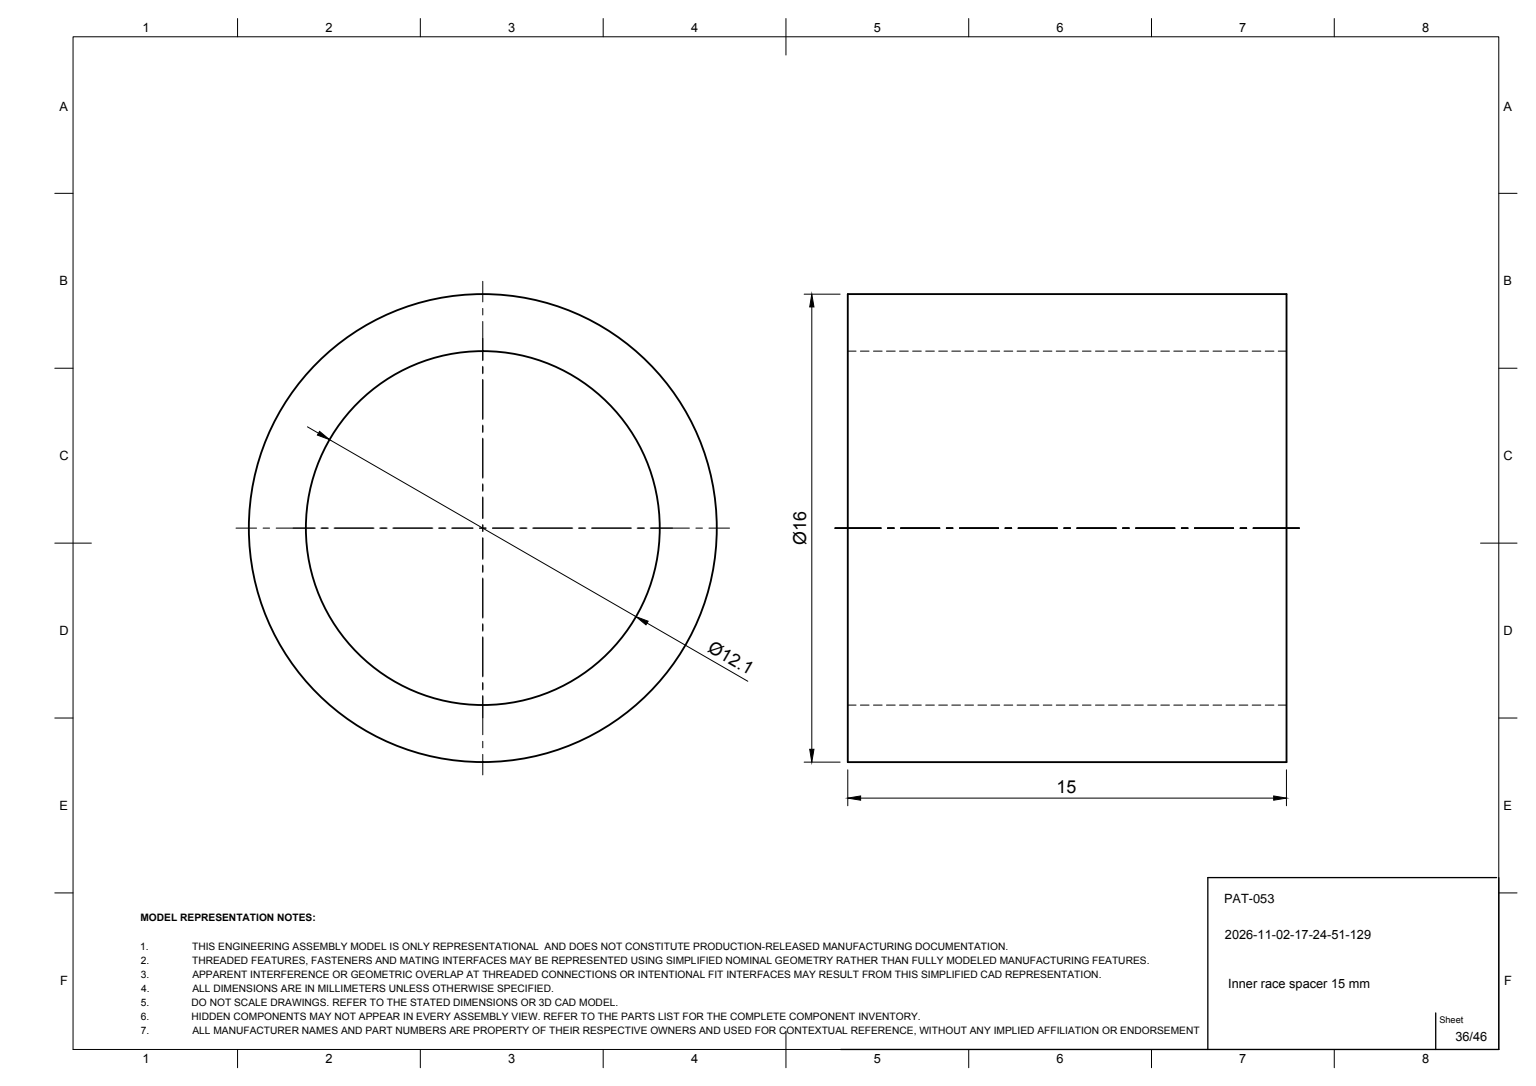
ISO-10303-21;
HEADER;
/* Generated by software containing ST-Developer
 * from STEP Tools, Inc. (www.steptools.com) 
 */

FILE_DESCRIPTION(
/* description */ ('Hand-operated arbor press'),
/* implementation_level */ '2;1');

FILE_NAME(
/* name */ 'Inner race spacer 15 mm.step',
/* time_stamp */ '2026-10-28T03:25:25-07:00',
/* author */ (''),
/* organization */ (''),
/* preprocessor_version */ 'ST-DEVELOPER v20.2',
/* originating_system */ 'Autodesk Translation Framework v15.17.0.0',
/* authorisation */ '');

FILE_SCHEMA (('AUTOMOTIVE_DESIGN { 1 0 10303 214 3 1 1 }'));
ENDSEC;

DATA;
#10=MECHANICAL_DESIGN_GEOMETRIC_PRESENTATION_REPRESENTATION('',(#621),#32751);
#530=SHAPE_REPRESENTATION_RELATIONSHIP('SRR','None',#32962,#572);
#572=ADVANCED_BREP_SHAPE_REPRESENTATION('',(#668),#32736);
#621=STYLED_ITEM('',(#33242),#668);
#668=MANIFOLD_SOLID_BREP('Body1',#12520);
#823=FACE_BOUND('',#2622,.T.);
#824=FACE_BOUND('',#2624,.T.);
#1208=PLANE('',#13838);
#1209=PLANE('',#13839);
#1795=FACE_OUTER_BOUND('',#2619,.T.);
#1796=FACE_OUTER_BOUND('',#2620,.T.);
#1797=FACE_OUTER_BOUND('',#2621,.T.);
#1798=FACE_OUTER_BOUND('',#2623,.T.);
#2619=EDGE_LOOP('',(#10800,#10801,#10802,#10803));
#2620=EDGE_LOOP('',(#10804,#10805,#10806,#10807));
#2621=EDGE_LOOP('',(#10808));
#2622=EDGE_LOOP('',(#10809));
#2623=EDGE_LOOP('',(#10810));
#2624=EDGE_LOOP('',(#10811));
#3756=LINE('',#20618,#4927);
#3757=LINE('',#20624,#4928);
#4927=VECTOR('',#16757,0.605);
#4928=VECTOR('',#16764,0.8);
#5454=CIRCLE('',#13833,0.605);
#5455=CIRCLE('',#13834,0.605);
#5456=CIRCLE('',#13836,0.8);
#5457=CIRCLE('',#13837,0.8);
#6387=VERTEX_POINT('',#20615);
#6388=VERTEX_POINT('',#20617);
#6389=VERTEX_POINT('',#20621);
#6390=VERTEX_POINT('',#20623);
#7903=EDGE_CURVE('',#6387,#6387,#5454,.T.);
#7904=EDGE_CURVE('',#6387,#6388,#3756,.T.);
#7905=EDGE_CURVE('',#6388,#6388,#5455,.T.);
#7906=EDGE_CURVE('',#6389,#6389,#5456,.T.);
#7907=EDGE_CURVE('',#6389,#6390,#3757,.T.);
#7908=EDGE_CURVE('',#6390,#6390,#5457,.T.);
#10800=ORIENTED_EDGE('',*,*,#7903,.F.);
#10801=ORIENTED_EDGE('',*,*,#7904,.T.);
#10802=ORIENTED_EDGE('',*,*,#7905,.T.);
#10803=ORIENTED_EDGE('',*,*,#7904,.F.);
#10804=ORIENTED_EDGE('',*,*,#7906,.F.);
#10805=ORIENTED_EDGE('',*,*,#7907,.T.);
#10806=ORIENTED_EDGE('',*,*,#7908,.T.);
#10807=ORIENTED_EDGE('',*,*,#7907,.F.);
#10808=ORIENTED_EDGE('',*,*,#7906,.T.);
#10809=ORIENTED_EDGE('',*,*,#7903,.T.);
#10810=ORIENTED_EDGE('',*,*,#7908,.F.);
#10811=ORIENTED_EDGE('',*,*,#7905,.F.);
#11756=CYLINDRICAL_SURFACE('',#13832,0.605);
#11757=CYLINDRICAL_SURFACE('',#13835,0.8);
#12304=ADVANCED_FACE('',(#1795),#11756,.F.);
#12305=ADVANCED_FACE('',(#1796),#11757,.T.);
#12306=ADVANCED_FACE('',(#1797,#823),#1208,.T.);
#12307=ADVANCED_FACE('',(#1798,#824),#1209,.F.);
#12520=CLOSED_SHELL('',(#12304,#12305,#12306,#12307));
#13831=AXIS2_PLACEMENT_3D('',#20613,#16751,#16752);
#13832=AXIS2_PLACEMENT_3D('',#20614,#16753,#16754);
#13833=AXIS2_PLACEMENT_3D('',#20616,#16755,#16756);
#13834=AXIS2_PLACEMENT_3D('',#20619,#16758,#16759);
#13835=AXIS2_PLACEMENT_3D('',#20620,#16760,#16761);
#13836=AXIS2_PLACEMENT_3D('',#20622,#16762,#16763);
#13837=AXIS2_PLACEMENT_3D('',#20625,#16765,#16766);
#13838=AXIS2_PLACEMENT_3D('',#20626,#16767,#16768);
#13839=AXIS2_PLACEMENT_3D('',#20627,#16769,#16770);
#16751=DIRECTION('axis',(0.,0.,1.));
#16752=DIRECTION('refdir',(1.,0.,0.));
#16753=DIRECTION('center_axis',(0.,1.,0.));
#16754=DIRECTION('ref_axis',(1.,0.,0.));
#16755=DIRECTION('center_axis',(0.,-1.,0.));
#16756=DIRECTION('ref_axis',(1.,0.,0.));
#16757=DIRECTION('',(0.,-1.,0.));
#16758=DIRECTION('center_axis',(0.,-1.,0.));
#16759=DIRECTION('ref_axis',(1.,0.,0.));
#16760=DIRECTION('center_axis',(0.,1.,0.));
#16761=DIRECTION('ref_axis',(1.,0.,0.));
#16762=DIRECTION('center_axis',(0.,1.,0.));
#16763=DIRECTION('ref_axis',(1.,0.,0.));
#16764=DIRECTION('',(0.,-1.,0.));
#16765=DIRECTION('center_axis',(0.,1.,0.));
#16766=DIRECTION('ref_axis',(1.,0.,0.));
#16767=DIRECTION('center_axis',(0.,1.,0.));
#16768=DIRECTION('ref_axis',(1.,0.,0.));
#16769=DIRECTION('center_axis',(0.,1.,0.));
#16770=DIRECTION('ref_axis',(1.,0.,0.));
#20613=CARTESIAN_POINT('',(0.,0.,0.));
#20614=CARTESIAN_POINT('Origin',(-3.25,-2.5,20.));
#20615=CARTESIAN_POINT('',(-3.855,-1.,20.));
#20616=CARTESIAN_POINT('Origin',(-3.25,-1.,20.));
#20617=CARTESIAN_POINT('',(-3.855,-2.5,20.));
#20618=CARTESIAN_POINT('',(-3.855,-2.5,20.));
#20619=CARTESIAN_POINT('Origin',(-3.25,-2.5,20.));
#20620=CARTESIAN_POINT('Origin',(-3.25,-2.5,20.));
#20621=CARTESIAN_POINT('',(-4.05,-1.,20.));
#20622=CARTESIAN_POINT('Origin',(-3.25,-1.,20.));
#20623=CARTESIAN_POINT('',(-4.05,-2.5,20.));
#20624=CARTESIAN_POINT('',(-4.05,-2.5,20.));
#20625=CARTESIAN_POINT('Origin',(-3.25,-2.5,20.));
#20626=CARTESIAN_POINT('Origin',(-3.25,-1.,20.));
#20627=CARTESIAN_POINT('Origin',(-3.25,-2.5,20.));
#32687=UNCERTAINTY_MEASURE_WITH_UNIT(LENGTH_MEASURE(0.001),#32752,
'DISTANCE_ACCURACY_VALUE',
'Maximum model space distance between geometric entities at asserted c
onnectivities');
#32702=UNCERTAINTY_MEASURE_WITH_UNIT(LENGTH_MEASURE(0.001),#32752,
'DISTANCE_ACCURACY_VALUE',
'Maximum model space distance between geometric entities at asserted c
onnectivities');
#32736=(
GEOMETRIC_REPRESENTATION_CONTEXT(3)
GLOBAL_UNCERTAINTY_ASSIGNED_CONTEXT((#32687))
GLOBAL_UNIT_ASSIGNED_CONTEXT((#32752,#32754,#32755))
REPRESENTATION_CONTEXT('','3D')
);
#32751=(
GEOMETRIC_REPRESENTATION_CONTEXT(3)
GLOBAL_UNCERTAINTY_ASSIGNED_CONTEXT((#32702))
GLOBAL_UNIT_ASSIGNED_CONTEXT((#32752,#32754,#32755))
REPRESENTATION_CONTEXT('','3D')
);
#32752=(
LENGTH_UNIT()
NAMED_UNIT(*)
SI_UNIT(.CENTI.,.METRE.)
);
#32754=(
NAMED_UNIT(*)
PLANE_ANGLE_UNIT()
SI_UNIT($,.RADIAN.)
);
#32755=(
NAMED_UNIT(*)
SI_UNIT($,.STERADIAN.)
SOLID_ANGLE_UNIT()
);
#32789=SHAPE_DEFINITION_REPRESENTATION(#32846,#32962);
#32846=PRODUCT_DEFINITION_SHAPE('',$,#33011);
#32962=SHAPE_REPRESENTATION('',(#13831),#32736);
#32977=PRODUCT_DEFINITION_CONTEXT('part definition',#33123,'design');
#33011=PRODUCT_DEFINITION('Inner race spacer 15 mm',
'Inner race spacer 15 mm',#33059,#32977);
#33059=PRODUCT_DEFINITION_FORMATION('',$,#33158);
#33123=APPLICATION_CONTEXT(
'Core Data for Automotive Mechanical Design Process');
#33124=PRODUCT_CONTEXT('part definition',#33123,'mechanical');
#33158=PRODUCT('Inner race spacer 15 mm','Inner race spacer 15 mm',
'Inner race spacer 15 mm',(#33124));
#33236=COLOUR_RGB('Grey',0.48,0.52,0.57);
#33237=FILL_AREA_STYLE_COLOUR('',#33236);
#33238=FILL_AREA_STYLE('',(#33237));
#33239=SURFACE_STYLE_FILL_AREA(#33238);
#33240=SURFACE_SIDE_STYLE('',(#33239));
#33241=SURFACE_STYLE_USAGE(.BOTH.,#33240);
#33242=PRESENTATION_STYLE_ASSIGNMENT((#33241));
ENDSEC;
END-ISO-10303-21;
